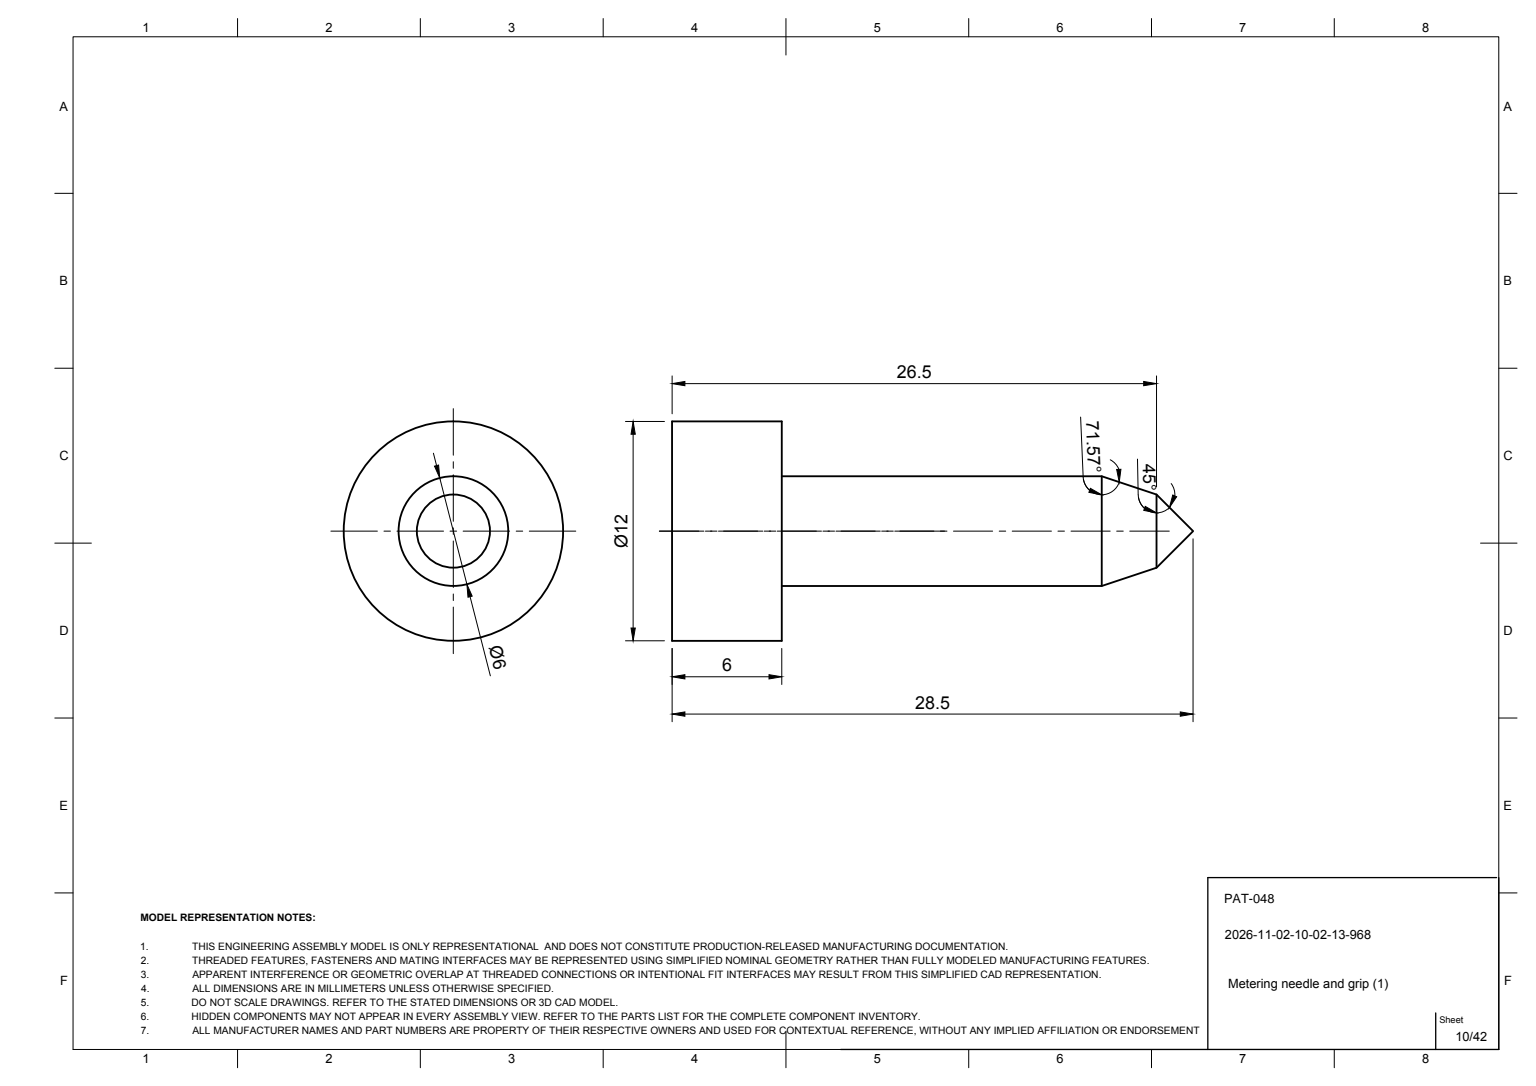
ISO-10303-21;
HEADER;
/* Generated by software containing ST-Developer
 * from STEP Tools, Inc. (www.steptools.com) 
 */

FILE_DESCRIPTION(
/* description */ ('Guided pneumatic stop gate'),
/* implementation_level */ '2;1');

FILE_NAME(
/* name */ 'Metering needle and grip (1).step',
/* time_stamp */ '2026-10-27T21:43:45-07:00',
/* author */ (''),
/* organization */ (''),
/* preprocessor_version */ 'ST-DEVELOPER v20.2',
/* originating_system */ 'Autodesk Translation Framework v15.17.0.0',
/* authorisation */ '');

FILE_SCHEMA (('AUTOMOTIVE_DESIGN { 1 0 10303 214 3 1 1 }'));
ENDSEC;

DATA;
#10=MECHANICAL_DESIGN_GEOMETRIC_PRESENTATION_REPRESENTATION('',(#540),#14392);
#425=CONICAL_SURFACE('',#8624,0.1,0.78539816339745);
#426=CONICAL_SURFACE('',#8626,0.25,0.321750554396641);
#456=SHAPE_REPRESENTATION_RELATIONSHIP('SRR','None',#14590,#498);
#498=ADVANCED_BREP_SHAPE_REPRESENTATION('',(#582),#14352);
#540=STYLED_ITEM('',(#14898),#582);
#582=MANIFOLD_SOLID_BREP('Body1',#7880);
#662=FACE_BOUND('',#1771,.T.);
#919=PLANE('',#8630);
#920=PLANE('',#8634);
#1245=FACE_OUTER_BOUND('',#1767,.T.);
#1246=FACE_OUTER_BOUND('',#1768,.T.);
#1247=FACE_OUTER_BOUND('',#1769,.T.);
#1248=FACE_OUTER_BOUND('',#1770,.T.);
#1249=FACE_OUTER_BOUND('',#1772,.T.);
#1250=FACE_OUTER_BOUND('',#1773,.T.);
#1767=EDGE_LOOP('',(#5844,#5845,#5846));
#1768=EDGE_LOOP('',(#5847,#5848,#5849,#5850));
#1769=EDGE_LOOP('',(#5851,#5852,#5853,#5854));
#1770=EDGE_LOOP('',(#5855));
#1771=EDGE_LOOP('',(#5856));
#1772=EDGE_LOOP('',(#5857,#5858,#5859,#5860));
#1773=EDGE_LOOP('',(#5861));
#2437=LINE('',#12487,#2982);
#2438=LINE('',#12491,#2983);
#2439=LINE('',#12495,#2984);
#2440=LINE('',#12502,#2985);
#2982=VECTOR('',#10024,0.1);
#2983=VECTOR('',#10029,0.25);
#2984=VECTOR('',#10034,0.3);
#2985=VECTOR('',#10043,0.6);
#3459=CIRCLE('',#8625,0.2);
#3460=CIRCLE('',#8627,0.3);
#3461=CIRCLE('',#8629,0.3);
#3462=CIRCLE('',#8631,0.6);
#3463=CIRCLE('',#8633,0.6);
#3901=VERTEX_POINT('',#12484);
#3902=VERTEX_POINT('',#12486);
#3903=VERTEX_POINT('',#12489);
#3904=VERTEX_POINT('',#12493);
#3905=VERTEX_POINT('',#12497);
#3906=VERTEX_POINT('',#12500);
#4620=EDGE_CURVE('',#3901,#3901,#3459,.T.);
#4621=EDGE_CURVE('',#3901,#3902,#2437,.T.);
#4622=EDGE_CURVE('',#3903,#3903,#3460,.T.);
#4623=EDGE_CURVE('',#3903,#3901,#2438,.T.);
#4624=EDGE_CURVE('',#3904,#3904,#3461,.T.);
#4625=EDGE_CURVE('',#3904,#3903,#2439,.T.);
#4626=EDGE_CURVE('',#3905,#3905,#3462,.T.);
#4627=EDGE_CURVE('',#3906,#3906,#3463,.T.);
#4628=EDGE_CURVE('',#3906,#3905,#2440,.T.);
#5844=ORIENTED_EDGE('',*,*,#4620,.F.);
#5845=ORIENTED_EDGE('',*,*,#4621,.T.);
#5846=ORIENTED_EDGE('',*,*,#4621,.F.);
#5847=ORIENTED_EDGE('',*,*,#4622,.F.);
#5848=ORIENTED_EDGE('',*,*,#4623,.T.);
#5849=ORIENTED_EDGE('',*,*,#4620,.T.);
#5850=ORIENTED_EDGE('',*,*,#4623,.F.);
#5851=ORIENTED_EDGE('',*,*,#4624,.F.);
#5852=ORIENTED_EDGE('',*,*,#4625,.T.);
#5853=ORIENTED_EDGE('',*,*,#4622,.T.);
#5854=ORIENTED_EDGE('',*,*,#4625,.F.);
#5855=ORIENTED_EDGE('',*,*,#4626,.F.);
#5856=ORIENTED_EDGE('',*,*,#4624,.T.);
#5857=ORIENTED_EDGE('',*,*,#4627,.F.);
#5858=ORIENTED_EDGE('',*,*,#4628,.T.);
#5859=ORIENTED_EDGE('',*,*,#4626,.T.);
#5860=ORIENTED_EDGE('',*,*,#4628,.F.);
#5861=ORIENTED_EDGE('',*,*,#4627,.T.);
#7281=CYLINDRICAL_SURFACE('',#8628,0.3);
#7282=CYLINDRICAL_SURFACE('',#8632,0.6);
#7527=ADVANCED_FACE('',(#1245),#425,.T.);
#7528=ADVANCED_FACE('',(#1246),#426,.T.);
#7529=ADVANCED_FACE('',(#1247),#7281,.T.);
#7530=ADVANCED_FACE('',(#1248,#662),#919,.T.);
#7531=ADVANCED_FACE('',(#1249),#7282,.T.);
#7532=ADVANCED_FACE('',(#1250),#920,.T.);
#7880=CLOSED_SHELL('',(#7527,#7528,#7529,#7530,#7531,#7532));
#8623=AXIS2_PLACEMENT_3D('',#12482,#10018,#10019);
#8624=AXIS2_PLACEMENT_3D('',#12483,#10020,#10021);
#8625=AXIS2_PLACEMENT_3D('',#12485,#10022,#10023);
#8626=AXIS2_PLACEMENT_3D('',#12488,#10025,#10026);
#8627=AXIS2_PLACEMENT_3D('',#12490,#10027,#10028);
#8628=AXIS2_PLACEMENT_3D('',#12492,#10030,#10031);
#8629=AXIS2_PLACEMENT_3D('',#12494,#10032,#10033);
#8630=AXIS2_PLACEMENT_3D('',#12496,#10035,#10036);
#8631=AXIS2_PLACEMENT_3D('',#12498,#10037,#10038);
#8632=AXIS2_PLACEMENT_3D('',#12499,#10039,#10040);
#8633=AXIS2_PLACEMENT_3D('',#12501,#10041,#10042);
#8634=AXIS2_PLACEMENT_3D('',#12503,#10044,#10045);
#10018=DIRECTION('axis',(0.,0.,1.));
#10019=DIRECTION('refdir',(1.,0.,0.));
#10020=DIRECTION('center_axis',(0.,0.,1.));
#10021=DIRECTION('ref_axis',(1.,0.,0.));
#10022=DIRECTION('center_axis',(0.,0.,1.));
#10023=DIRECTION('ref_axis',(1.,0.,0.));
#10024=DIRECTION('',(0.707106781186549,8.65956056235495E-17,-0.707106781186546));
#10025=DIRECTION('center_axis',(0.,0.,1.));
#10026=DIRECTION('ref_axis',(1.,0.,0.));
#10027=DIRECTION('center_axis',(0.,0.,1.));
#10028=DIRECTION('ref_axis',(1.,0.,0.));
#10029=DIRECTION('',(0.316227766016837,3.87267321454038E-17,-0.948683298050514));
#10030=DIRECTION('center_axis',(0.,0.,1.));
#10031=DIRECTION('ref_axis',(1.,0.,0.));
#10032=DIRECTION('center_axis',(0.,0.,1.));
#10033=DIRECTION('ref_axis',(1.,0.,0.));
#10034=DIRECTION('',(0.,0.,-1.));
#10035=DIRECTION('center_axis',(0.,0.,-1.));
#10036=DIRECTION('ref_axis',(-1.,0.,0.));
#10037=DIRECTION('center_axis',(0.,0.,1.));
#10038=DIRECTION('ref_axis',(1.,0.,0.));
#10039=DIRECTION('center_axis',(0.,0.,1.));
#10040=DIRECTION('ref_axis',(1.,0.,0.));
#10041=DIRECTION('center_axis',(0.,0.,1.));
#10042=DIRECTION('ref_axis',(1.,0.,0.));
#10043=DIRECTION('',(0.,0.,-1.));
#10044=DIRECTION('center_axis',(0.,0.,1.));
#10045=DIRECTION('ref_axis',(1.,0.,0.));
#12482=CARTESIAN_POINT('',(0.,0.,0.));
#12483=CARTESIAN_POINT('Origin',(0.,11.8,8.15));
#12484=CARTESIAN_POINT('',(-0.2,11.8,8.25));
#12485=CARTESIAN_POINT('Origin',(0.,11.8,8.25));
#12486=CARTESIAN_POINT('',(0.,11.8,8.05));
#12487=CARTESIAN_POINT('',(-0.1,11.8,8.15));
#12488=CARTESIAN_POINT('Origin',(0.,11.8,8.4));
#12489=CARTESIAN_POINT('',(-0.3,11.8,8.55));
#12490=CARTESIAN_POINT('Origin',(0.,11.8,8.55));
#12491=CARTESIAN_POINT('',(-0.25,11.8,8.4));
#12492=CARTESIAN_POINT('Origin',(0.,11.8,9.425));
#12493=CARTESIAN_POINT('',(-0.3,11.8,10.3));
#12494=CARTESIAN_POINT('Origin',(0.,11.8,10.3));
#12495=CARTESIAN_POINT('',(-0.3,11.8,9.425));
#12496=CARTESIAN_POINT('Origin',(0.6,11.8,10.3));
#12497=CARTESIAN_POINT('',(-0.6,11.8,10.3));
#12498=CARTESIAN_POINT('Origin',(0.,11.8,10.3));
#12499=CARTESIAN_POINT('Origin',(0.,11.8,10.6));
#12500=CARTESIAN_POINT('',(-0.6,11.8,10.9));
#12501=CARTESIAN_POINT('Origin',(0.,11.8,10.9));
#12502=CARTESIAN_POINT('',(-0.6,11.8,10.6));
#12503=CARTESIAN_POINT('Origin',(0.,11.8,10.9));
#14304=UNCERTAINTY_MEASURE_WITH_UNIT(LENGTH_MEASURE(0.001),#14393,
'DISTANCE_ACCURACY_VALUE',
'Maximum model space distance between geometric entities at asserted c
onnectivities');
#14344=UNCERTAINTY_MEASURE_WITH_UNIT(LENGTH_MEASURE(0.001),#14393,
'DISTANCE_ACCURACY_VALUE',
'Maximum model space distance between geometric entities at asserted c
onnectivities');
#14352=(
GEOMETRIC_REPRESENTATION_CONTEXT(3)
GLOBAL_UNCERTAINTY_ASSIGNED_CONTEXT((#14304))
GLOBAL_UNIT_ASSIGNED_CONTEXT((#14393,#14395,#14396))
REPRESENTATION_CONTEXT('','3D')
);
#14392=(
GEOMETRIC_REPRESENTATION_CONTEXT(3)
GLOBAL_UNCERTAINTY_ASSIGNED_CONTEXT((#14344))
GLOBAL_UNIT_ASSIGNED_CONTEXT((#14393,#14395,#14396))
REPRESENTATION_CONTEXT('','3D')
);
#14393=(
LENGTH_UNIT()
NAMED_UNIT(*)
SI_UNIT(.CENTI.,.METRE.)
);
#14395=(
NAMED_UNIT(*)
PLANE_ANGLE_UNIT()
SI_UNIT($,.RADIAN.)
);
#14396=(
NAMED_UNIT(*)
SI_UNIT($,.STERADIAN.)
SOLID_ANGLE_UNIT()
);
#14404=SHAPE_DEFINITION_REPRESENTATION(#14451,#14590);
#14451=PRODUCT_DEFINITION_SHAPE('',$,#14638);
#14590=SHAPE_REPRESENTATION('',(#8623),#14352);
#14630=PRODUCT_DEFINITION_CONTEXT('part definition',#14773,'design');
#14638=PRODUCT_DEFINITION('Metering needle and grip (1)',
'Metering needle and grip (1)',#14685,#14630);
#14685=PRODUCT_DEFINITION_FORMATION('',$,#14782);
#14773=APPLICATION_CONTEXT(
'Core Data for Automotive Mechanical Design Process');
#14774=PRODUCT_CONTEXT('part definition',#14773,'mechanical');
#14782=PRODUCT('Metering needle and grip (1)',
'Metering needle and grip (1)','Metering needle and grip (1)',(#14774));
#14892=COLOUR_RGB('Black',0.12,0.14,0.17);
#14893=FILL_AREA_STYLE_COLOUR('',#14892);
#14894=FILL_AREA_STYLE('',(#14893));
#14895=SURFACE_STYLE_FILL_AREA(#14894);
#14896=SURFACE_SIDE_STYLE('',(#14895));
#14897=SURFACE_STYLE_USAGE(.BOTH.,#14896);
#14898=PRESENTATION_STYLE_ASSIGNMENT((#14897));
ENDSEC;
END-ISO-10303-21;
